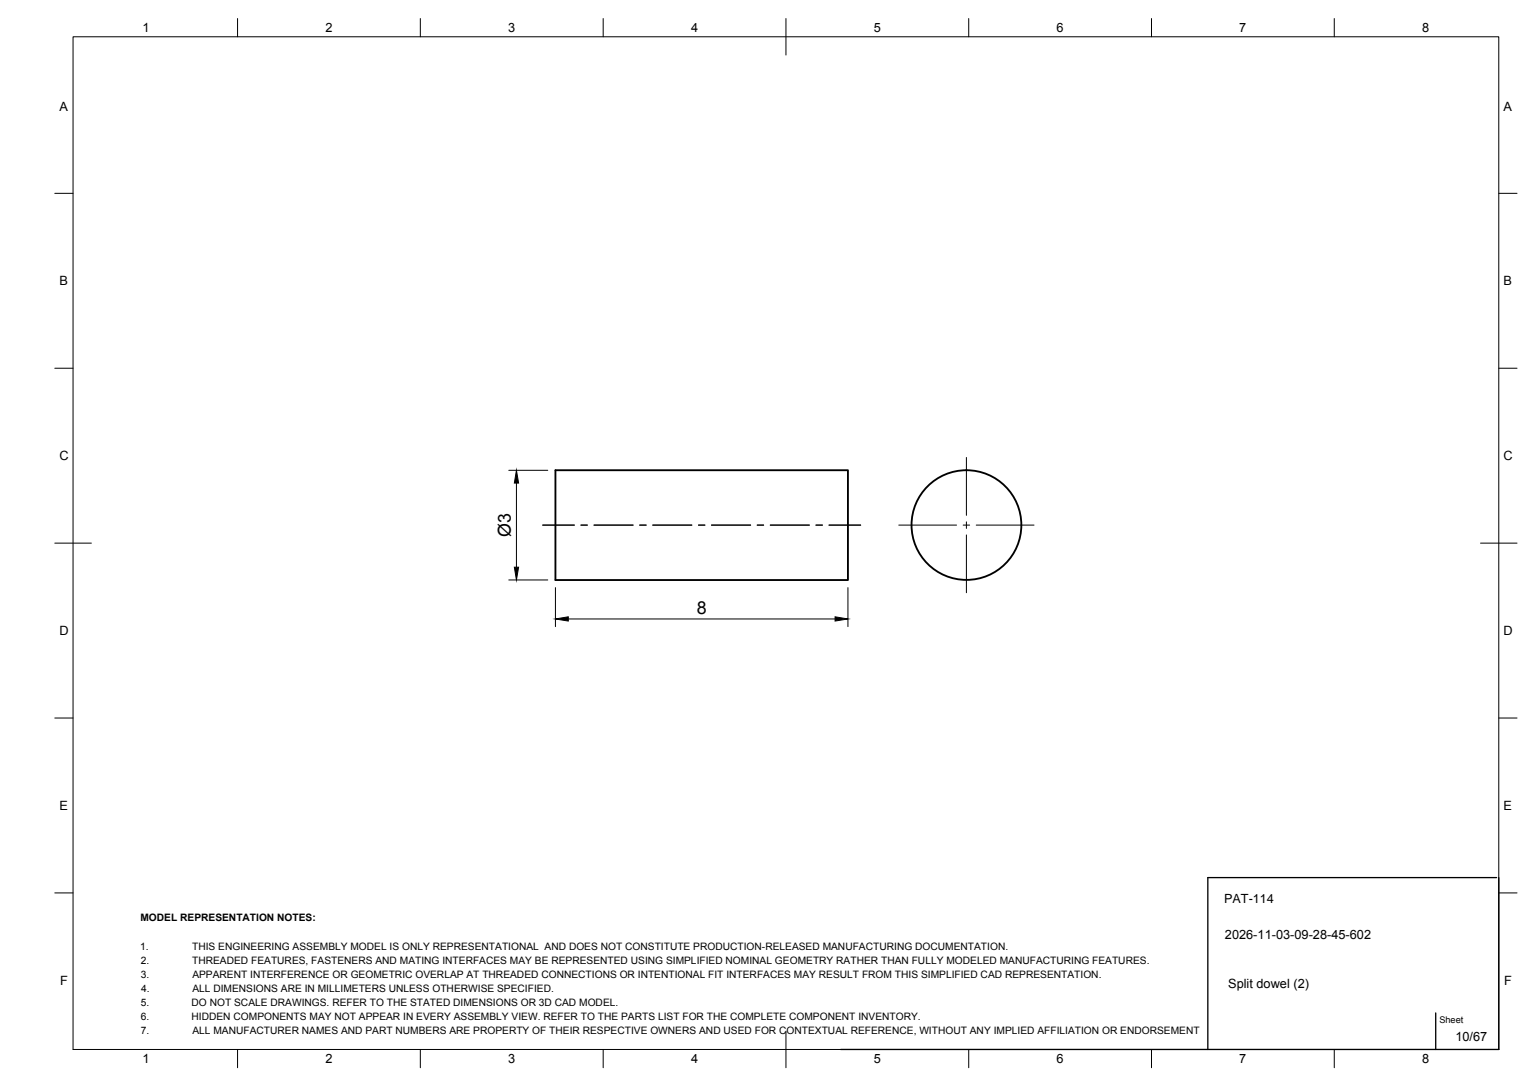
ISO-10303-21;
HEADER;
/* Generated by software containing ST-Developer
 * from STEP Tools, Inc. (www.steptools.com) 
 */

FILE_DESCRIPTION(
/* description */ ('Two-stage gear reducer in split housing'),
/* implementation_level */ '2;1');

FILE_NAME(
/* name */ 'Split dowel (2).step',
/* time_stamp */ '2026-10-28T03:22:31-07:00',
/* author */ (''),
/* organization */ (''),
/* preprocessor_version */ 'ST-DEVELOPER v20.2',
/* originating_system */ 'Autodesk Translation Framework v15.17.0.0',
/* authorisation */ '');

FILE_SCHEMA (('AUTOMOTIVE_DESIGN { 1 0 10303 214 3 1 1 }'));
ENDSEC;

DATA;
#10=MECHANICAL_DESIGN_GEOMETRIC_PRESENTATION_REPRESENTATION('',(#1239),#73366);
#1127=SHAPE_REPRESENTATION_RELATIONSHIP('SRR','None',#73614,#1183);
#1183=ADVANCED_BREP_SHAPE_REPRESENTATION('',(#1310),#73310);
#1239=STYLED_ITEM('',(#73974),#1310);
#1310=MANIFOLD_SOLID_BREP('Body1',#16127);
#1704=PLANE('',#17183);
#1705=PLANE('',#17184);
#2190=FACE_OUTER_BOUND('',#3189,.T.);
#2191=FACE_OUTER_BOUND('',#3190,.T.);
#2192=FACE_OUTER_BOUND('',#3191,.T.);
#3189=EDGE_LOOP('',(#11359,#11360,#11361,#11362));
#3190=EDGE_LOOP('',(#11363));
#3191=EDGE_LOOP('',(#11364));
#4310=LINE('',#23684,#5334);
#5334=VECTOR('',#19452,0.149999999999999);
#6276=CIRCLE('',#17181,0.149999999999999);
#6277=CIRCLE('',#17182,0.149999999999999);
#7108=VERTEX_POINT('',#23681);
#7109=VERTEX_POINT('',#23683);
#8733=EDGE_CURVE('',#7108,#7108,#6276,.T.);
#8734=EDGE_CURVE('',#7108,#7109,#4310,.T.);
#8735=EDGE_CURVE('',#7109,#7109,#6277,.T.);
#11359=ORIENTED_EDGE('',*,*,#8733,.F.);
#11360=ORIENTED_EDGE('',*,*,#8734,.T.);
#11361=ORIENTED_EDGE('',*,*,#8735,.T.);
#11362=ORIENTED_EDGE('',*,*,#8734,.F.);
#11363=ORIENTED_EDGE('',*,*,#8733,.T.);
#11364=ORIENTED_EDGE('',*,*,#8735,.F.);
#14993=CYLINDRICAL_SURFACE('',#17180,0.149999999999999);
#15397=ADVANCED_FACE('',(#2190),#14993,.T.);
#15398=ADVANCED_FACE('',(#2191),#1704,.T.);
#15399=ADVANCED_FACE('',(#2192),#1705,.F.);
#16127=CLOSED_SHELL('',(#15397,#15398,#15399));
#17179=AXIS2_PLACEMENT_3D('',#23679,#19446,#19447);
#17180=AXIS2_PLACEMENT_3D('',#23680,#19448,#19449);
#17181=AXIS2_PLACEMENT_3D('',#23682,#19450,#19451);
#17182=AXIS2_PLACEMENT_3D('',#23685,#19453,#19454);
#17183=AXIS2_PLACEMENT_3D('',#23686,#19455,#19456);
#17184=AXIS2_PLACEMENT_3D('',#23687,#19457,#19458);
#19446=DIRECTION('axis',(0.,0.,1.));
#19447=DIRECTION('refdir',(1.,0.,0.));
#19448=DIRECTION('center_axis',(0.,0.,1.));
#19449=DIRECTION('ref_axis',(1.,0.,0.));
#19450=DIRECTION('center_axis',(0.,0.,1.));
#19451=DIRECTION('ref_axis',(1.,0.,0.));
#19452=DIRECTION('',(0.,0.,-1.));
#19453=DIRECTION('center_axis',(0.,0.,1.));
#19454=DIRECTION('ref_axis',(1.,0.,0.));
#19455=DIRECTION('center_axis',(0.,0.,1.));
#19456=DIRECTION('ref_axis',(1.,0.,0.));
#19457=DIRECTION('center_axis',(0.,0.,1.));
#19458=DIRECTION('ref_axis',(1.,0.,0.));
#23679=CARTESIAN_POINT('',(0.,0.,0.));
#23680=CARTESIAN_POINT('Origin',(17.75,-3.,9.6));
#23681=CARTESIAN_POINT('',(17.6,-3.,10.4));
#23682=CARTESIAN_POINT('Origin',(17.75,-3.,10.4));
#23683=CARTESIAN_POINT('',(17.6,-3.,9.6));
#23684=CARTESIAN_POINT('',(17.6,-3.,9.6));
#23685=CARTESIAN_POINT('Origin',(17.75,-3.,9.6));
#23686=CARTESIAN_POINT('Origin',(17.75,-3.,10.4));
#23687=CARTESIAN_POINT('Origin',(17.75,-3.,9.6));
#73246=UNCERTAINTY_MEASURE_WITH_UNIT(LENGTH_MEASURE(0.001),#73367,
'DISTANCE_ACCURACY_VALUE',
'Maximum model space distance between geometric entities at asserted c
onnectivities');
#73302=UNCERTAINTY_MEASURE_WITH_UNIT(LENGTH_MEASURE(0.001),#73367,
'DISTANCE_ACCURACY_VALUE',
'Maximum model space distance between geometric entities at asserted c
onnectivities');
#73310=(
GEOMETRIC_REPRESENTATION_CONTEXT(3)
GLOBAL_UNCERTAINTY_ASSIGNED_CONTEXT((#73246))
GLOBAL_UNIT_ASSIGNED_CONTEXT((#73367,#73369,#73370))
REPRESENTATION_CONTEXT('','3D')
);
#73366=(
GEOMETRIC_REPRESENTATION_CONTEXT(3)
GLOBAL_UNCERTAINTY_ASSIGNED_CONTEXT((#73302))
GLOBAL_UNIT_ASSIGNED_CONTEXT((#73367,#73369,#73370))
REPRESENTATION_CONTEXT('','3D')
);
#73367=(
LENGTH_UNIT()
NAMED_UNIT(*)
SI_UNIT(.CENTI.,.METRE.)
);
#73369=(
NAMED_UNIT(*)
PLANE_ANGLE_UNIT()
SI_UNIT($,.RADIAN.)
);
#73370=(
NAMED_UNIT(*)
SI_UNIT($,.STERADIAN.)
SOLID_ANGLE_UNIT()
);
#73378=SHAPE_DEFINITION_REPRESENTATION(#73441,#73614);
#73441=PRODUCT_DEFINITION_SHAPE('',$,#73678);
#73614=SHAPE_REPRESENTATION('',(#17179),#73310);
#73670=PRODUCT_DEFINITION_CONTEXT('part definition',#73861,'design');
#73678=PRODUCT_DEFINITION('Split dowel (2)','Split dowel (2)',#73741,#73670);
#73741=PRODUCT_DEFINITION_FORMATION('',$,#73870);
#73861=APPLICATION_CONTEXT(
'Core Data for Automotive Mechanical Design Process');
#73862=PRODUCT_CONTEXT('part definition',#73861,'mechanical');
#73870=PRODUCT('Split dowel (2)','Split dowel (2)','Split dowel (2)',(#73862));
#73968=COLOUR_RGB('Light Blue',0.38,0.62,0.78);
#73969=FILL_AREA_STYLE_COLOUR('',#73968);
#73970=FILL_AREA_STYLE('',(#73969));
#73971=SURFACE_STYLE_FILL_AREA(#73970);
#73972=SURFACE_SIDE_STYLE('',(#73971));
#73973=SURFACE_STYLE_USAGE(.BOTH.,#73972);
#73974=PRESENTATION_STYLE_ASSIGNMENT((#73973));
ENDSEC;
END-ISO-10303-21;
